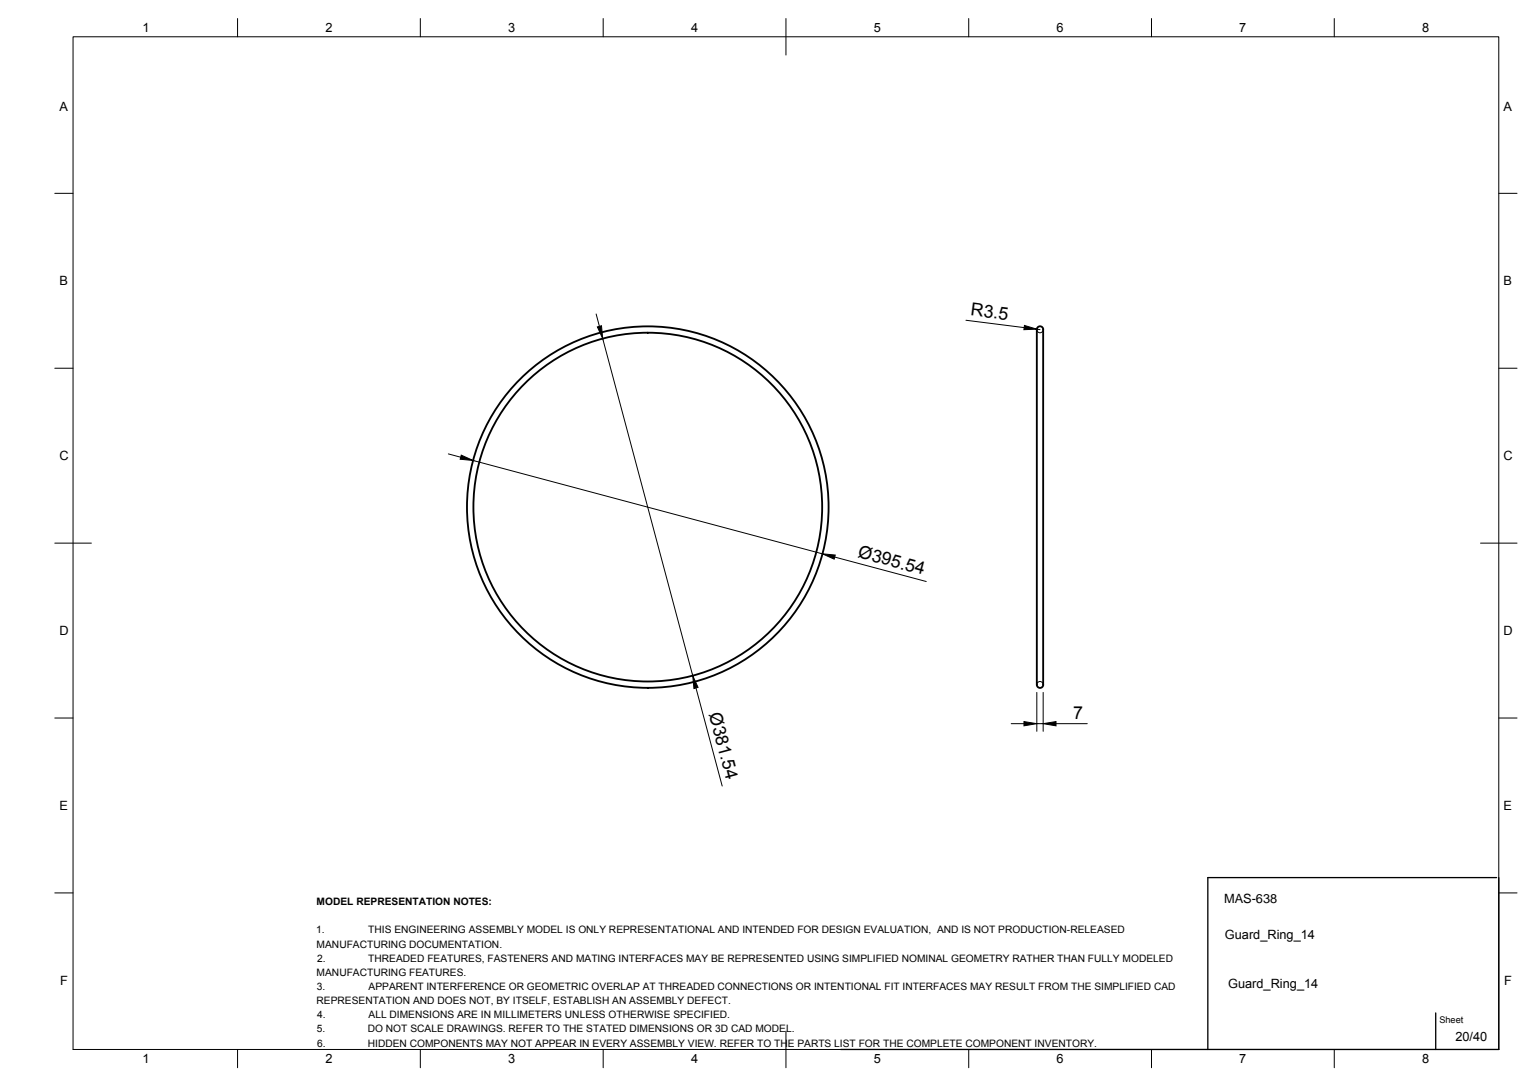
ISO-10303-21;
HEADER;
FILE_DESCRIPTION((''),'2;1');
FILE_NAME('Guard_Ring_14.step','2026-10-09T12:00:21-07:00',(''),(''),'','','');
FILE_SCHEMA (('AUTOMOTIVE_DESIGN { 1 0 10303 214 3 1 1 }'));
ENDSEC;
DATA;
#10=MECHANICAL_DESIGN_GEOMETRIC_PRESENTATION_REPRESENTATION('',(#417,#418),#10334);
#347=SHAPE_REPRESENTATION_RELATIONSHIP('SRR','None',#10463,#379) ;
#379=ADVANCED_BREP_SHAPE_REPRESENTATION('',(#451),#10315) ;
#417=STYLED_ITEM('',(#10631),#3380) ;
#418=STYLED_ITEM('',(#10632),#451) ;
#451=MANIFOLD_SOLID_BREP('Body1',#3573) ;
#872=FACE_OUTER_BOUND('',#1072,.T.) ;
#1072=EDGE_LOOP('',(#2401,#2402,#2403,#2404)) ;
#1302=CIRCLE('',#4027,0.349999999999999) ;
#1303=CIRCLE('',#4028,19.0768144613668) ;
#1526=VERTEX_POINT('',#5718) ;
#1857=EDGE_CURVE('',#1526,#1526,#1302,.T.) ;
#1858=EDGE_CURVE('',#1526,#1526,#1303,.T.) ;
#2401=ORIENTED_EDGE('',*,*,#1857,.F.) ;
#2402=ORIENTED_EDGE('',*,*,#1858,.T.) ;
#2403=ORIENTED_EDGE('',*,*,#1857,.T.) ;
#2404=ORIENTED_EDGE('',*,*,#1858,.F.) ;
#3318=TOROIDAL_SURFACE('',#4026,19.4268144613668,0.349999999999999) ;
#3380=ADVANCED_FACE('',(#872),#3318,.T.) ;
#3573=CLOSED_SHELL('',(#3380)) ;
#4025=AXIS2_PLACEMENT_3D('',#5716,#4611,#4612) ;
#4026=AXIS2_PLACEMENT_3D('',#5717,#4613,#4614) ;
#4027=AXIS2_PLACEMENT_3D('',#5719,#4615,#4616) ;
#4028=AXIS2_PLACEMENT_3D('',#5720,#4617,#4618) ;
#4611=DIRECTION('axis',(0.,0.,1.)) ;
#4612=DIRECTION('refdir',(1.,0.,0.)) ;
#4613=DIRECTION('center_axis',(-6.42891162084177E-17,-1.,-1.01883556321148E-16)) ;
#4614=DIRECTION('ref_axis',(1.,0.,0.)) ;
#4615=DIRECTION('center_axis',(0.,1.01883556321148E-16,-1.)) ;
#4616=DIRECTION('ref_axis',(-1.,0.,0.)) ;
#4617=DIRECTION('center_axis',(6.42891162084177E-17,1.,1.01883556321148E-16)) ;
#4618=DIRECTION('ref_axis',(1.,-6.42891162084177E-17,-6.55000379205715E-33)) ;
#5716=CARTESIAN_POINT('',(0.,0.,0.)) ;
#5717=CARTESIAN_POINT('Origin',(23.47768801576,67.3831179463143,68.2224337400009)) ;
#5718=CARTESIAN_POINT('',(4.4008735543932,67.3831179463143,68.2224337400009)) ;
#5719=CARTESIAN_POINT('Origin',(4.0508735543932,67.3831179463143,68.2224337400009)) ;
#5720=CARTESIAN_POINT('Origin',(23.47768801576,67.3831179463143,68.2224337400009)) ;
#10278=UNCERTAINTY_MEASURE_WITH_UNIT(LENGTH_MEASURE(0.001),#10335,
'DISTANCE_ACCURACY_VALUE',
'Maximum model space distance between geometric entities at asserted c
onnectivities') ;
#10297=UNCERTAINTY_MEASURE_WITH_UNIT(LENGTH_MEASURE(0.001),#10335,
'DISTANCE_ACCURACY_VALUE',
'Maximum model space distance between geometric entities at asserted c
onnectivities') ;
#10315=(
GEOMETRIC_REPRESENTATION_CONTEXT(3)
GLOBAL_UNCERTAINTY_ASSIGNED_CONTEXT((#10278))
GLOBAL_UNIT_ASSIGNED_CONTEXT((#10335,#10337,#10338))
REPRESENTATION_CONTEXT('','3D')
) ;
#10334=(
GEOMETRIC_REPRESENTATION_CONTEXT(3)
GLOBAL_UNCERTAINTY_ASSIGNED_CONTEXT((#10297))
GLOBAL_UNIT_ASSIGNED_CONTEXT((#10335,#10337,#10338))
REPRESENTATION_CONTEXT('','3D')
) ;
#10335=(
LENGTH_UNIT()
NAMED_UNIT(*)
SI_UNIT(.CENTI.,.METRE.)
) ;
#10337=(
NAMED_UNIT(*)
PLANE_ANGLE_UNIT()
SI_UNIT($,.RADIAN.)
) ;
#10338=(
NAMED_UNIT(*)
SI_UNIT($,.STERADIAN.)
SOLID_ANGLE_UNIT()
) ;
#10356=SHAPE_DEFINITION_REPRESENTATION(#10392,#10463) ;
#10392=PRODUCT_DEFINITION_SHAPE('',$,#10500) ;
#10463=SHAPE_REPRESENTATION('',(#4025),#10315) ;
#10482=PRODUCT_DEFINITION_CONTEXT('part definition',#10592,'design') ;
#10500=PRODUCT_DEFINITION('Guard_Ring_14','Guard_Ring_14',#10536,#10482) ;
#10536=PRODUCT_DEFINITION_FORMATION('',$,#10611) ;
#10592=APPLICATION_CONTEXT(
'Core Data for Automotive Mechanical Design Process') ;
#10593=PRODUCT_CONTEXT('part definition',#10592,'mechanical') ;
#10611=PRODUCT('Guard_Ring_14','Guard_Ring_14',$,(#10593)) ;
#10631=PRESENTATION_STYLE_ASSIGNMENT((#10635)) ;
#10632=PRESENTATION_STYLE_ASSIGNMENT((#10636)) ;
#10635=SURFACE_STYLE_USAGE(.BOTH.,#10639) ;
#10636=SURFACE_STYLE_USAGE(.BOTH.,#10640) ;
#10639=SURFACE_SIDE_STYLE('',(#10643)) ;
#10640=SURFACE_SIDE_STYLE('',(#10644)) ;
#10643=SURFACE_STYLE_FILL_AREA(#10647) ;
#10644=SURFACE_STYLE_FILL_AREA(#10648) ;
#10647=FILL_AREA_STYLE('Opaque(25,25,25)',(#10651)) ;
#10648=FILL_AREA_STYLE('Opaque(202,209,238)',(#10652)) ;
#10651=FILL_AREA_STYLE_COLOUR('Opaque(25,25,25)',#10655) ;
#10652=FILL_AREA_STYLE_COLOUR('Opaque(202,209,238)',#10656) ;
#10655=COLOUR_RGB('Opaque(25,25,25)', 0.09019608, 0.27058824, 0.51372549) ;
#10656=COLOUR_RGB('Opaque(202,209,238)', 0.40784314, 0.44705882, 0.49803922) ;
ENDSEC;
END-ISO-10303-21;
